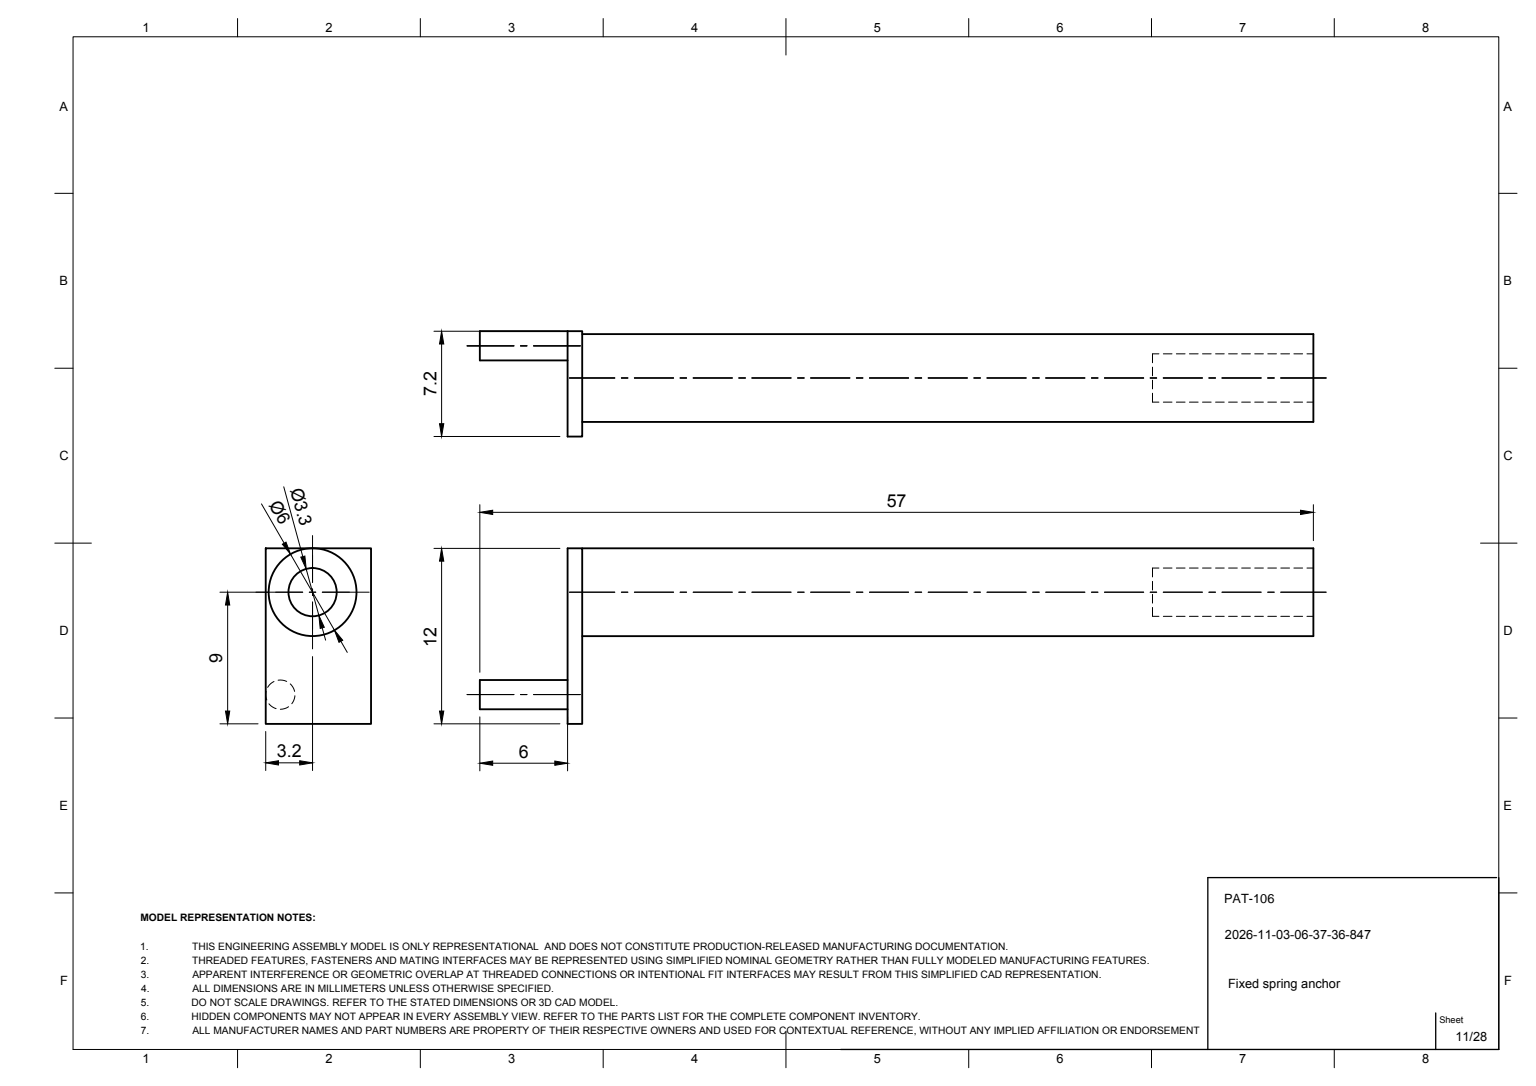
ISO-10303-21;
HEADER;
/* Generated by software containing ST-Developer
 * from STEP Tools, Inc. (www.steptools.com) 
 */

FILE_DESCRIPTION(
/* description */ ('Torsion-spring ratchet demonstrator'),
/* implementation_level */ '2;1');

FILE_NAME(
/* name */ 'Fixed spring anchor.step',
/* time_stamp */ '2026-10-29T17:29:17-07:00',
/* author */ (''),
/* organization */ (''),
/* preprocessor_version */ 'ST-DEVELOPER v20.2',
/* originating_system */ 'Autodesk Translation Framework v15.17.0.0',
/* authorisation */ '');

FILE_SCHEMA (('AUTOMOTIVE_DESIGN { 1 0 10303 214 3 1 1 }'));
ENDSEC;

DATA;
#10=MECHANICAL_DESIGN_GEOMETRIC_PRESENTATION_REPRESENTATION('',(#289),#11258);
#241=SHAPE_REPRESENTATION_RELATIONSHIP('SRR','None',#11367,#265);
#265=ADVANCED_BREP_SHAPE_REPRESENTATION('',(#321),#11237);
#289=STYLED_ITEM('',(#11584),#321);
#321=MANIFOLD_SOLID_BREP('Body1',#5160);
#375=FACE_BOUND('',#1015,.T.);
#461=PLANE('',#5552);
#462=PLANE('',#5557);
#463=PLANE('',#5558);
#464=PLANE('',#5559);
#465=PLANE('',#5562);
#466=PLANE('',#5563);
#467=PLANE('',#5564);
#468=PLANE('',#5565);
#469=PLANE('',#5568);
#668=FACE_OUTER_BOUND('',#1003,.T.);
#669=FACE_OUTER_BOUND('',#1004,.T.);
#670=FACE_OUTER_BOUND('',#1005,.T.);
#671=FACE_OUTER_BOUND('',#1006,.T.);
#672=FACE_OUTER_BOUND('',#1007,.T.);
#673=FACE_OUTER_BOUND('',#1008,.T.);
#674=FACE_OUTER_BOUND('',#1009,.T.);
#675=FACE_OUTER_BOUND('',#1010,.T.);
#676=FACE_OUTER_BOUND('',#1011,.T.);
#677=FACE_OUTER_BOUND('',#1012,.T.);
#678=FACE_OUTER_BOUND('',#1013,.T.);
#679=FACE_OUTER_BOUND('',#1014,.T.);
#1003=EDGE_LOOP('',(#3616,#3617,#3618,#3619));
#1004=EDGE_LOOP('',(#3620));
#1005=EDGE_LOOP('',(#3621,#3622,#3623,#3624,#3625));
#1006=EDGE_LOOP('',(#3626));
#1007=EDGE_LOOP('',(#3627,#3628,#3629,#3630,#3631,#3632,#3633));
#1008=EDGE_LOOP('',(#3634,#3635,#3636,#3637,#3638,#3639,#3640));
#1009=EDGE_LOOP('',(#3641,#3642,#3643,#3644));
#1010=EDGE_LOOP('',(#3645,#3646,#3647,#3648,#3649));
#1011=EDGE_LOOP('',(#3650,#3651,#3652,#3653,#3654));
#1012=EDGE_LOOP('',(#3655,#3656,#3657,#3658));
#1013=EDGE_LOOP('',(#3659,#3660,#3661,#3662,#3663));
#1014=EDGE_LOOP('',(#3664));
#1015=EDGE_LOOP('',(#3665));
#1370=LINE('',#7878,#1753);
#1371=LINE('',#7885,#1754);
#1372=LINE('',#7893,#1755);
#1373=LINE('',#7894,#1756);
#1374=LINE('',#7896,#1757);
#1375=LINE('',#7898,#1758);
#1376=LINE('',#7899,#1759);
#1377=LINE('',#7903,#1760);
#1378=LINE('',#7905,#1761);
#1379=LINE('',#7907,#1762);
#1380=LINE('',#7912,#1763);
#1381=LINE('',#7913,#1764);
#1382=LINE('',#7915,#1765);
#1383=LINE('',#7916,#1766);
#1384=LINE('',#7918,#1767);
#1385=LINE('',#7920,#1768);
#1386=LINE('',#7924,#1769);
#1753=VECTOR('',#6307,0.164999999999999);
#1754=VECTOR('',#6316,0.0999999999999996);
#1755=VECTOR('',#6325,1.);
#1756=VECTOR('',#6326,1.);
#1757=VECTOR('',#6327,1.);
#1758=VECTOR('',#6328,1.);
#1759=VECTOR('',#6329,1.);
#1760=VECTOR('',#6332,1.);
#1761=VECTOR('',#6333,1.);
#1762=VECTOR('',#6334,1.);
#1763=VECTOR('',#6339,1.);
#1764=VECTOR('',#6340,1.);
#1765=VECTOR('',#6343,1.);
#1766=VECTOR('',#6344,1.);
#1767=VECTOR('',#6347,1.);
#1768=VECTOR('',#6350,1.);
#1769=VECTOR('',#6355,0.300000000000001);
#2133=CIRCLE('',#5550,0.164999999999999);
#2134=CIRCLE('',#5551,0.164999999999999);
#2135=CIRCLE('',#5554,0.0999999999999996);
#2136=CIRCLE('',#5555,0.0999999999999996);
#2137=CIRCLE('',#5556,0.0999999999999996);
#2138=CIRCLE('',#5560,0.300000000000001);
#2139=CIRCLE('',#5561,0.300000000000001);
#2140=CIRCLE('',#5567,0.300000000000001);
#2393=VERTEX_POINT('',#7875);
#2394=VERTEX_POINT('',#7877);
#2395=VERTEX_POINT('',#7882);
#2396=VERTEX_POINT('',#7884);
#2397=VERTEX_POINT('',#7886);
#2398=VERTEX_POINT('',#7891);
#2399=VERTEX_POINT('',#7892);
#2400=VERTEX_POINT('',#7895);
#2401=VERTEX_POINT('',#7897);
#2402=VERTEX_POINT('',#7901);
#2403=VERTEX_POINT('',#7902);
#2404=VERTEX_POINT('',#7904);
#2405=VERTEX_POINT('',#7906);
#2406=VERTEX_POINT('',#7908);
#2407=VERTEX_POINT('',#7911);
#2408=VERTEX_POINT('',#7923);
#2868=EDGE_CURVE('',#2393,#2393,#2133,.T.);
#2869=EDGE_CURVE('',#2393,#2394,#1370,.T.);
#2870=EDGE_CURVE('',#2394,#2394,#2134,.T.);
#2871=EDGE_CURVE('',#2395,#2395,#2135,.T.);
#2872=EDGE_CURVE('',#2395,#2396,#1371,.T.);
#2873=EDGE_CURVE('',#2397,#2396,#2136,.T.);
#2874=EDGE_CURVE('',#2396,#2397,#2137,.T.);
#2875=EDGE_CURVE('',#2398,#2399,#1372,.T.);
#2876=EDGE_CURVE('',#2399,#2397,#1373,.T.);
#2877=EDGE_CURVE('',#2397,#2400,#1374,.T.);
#2878=EDGE_CURVE('',#2400,#2401,#1375,.T.);
#2879=EDGE_CURVE('',#2401,#2398,#1376,.T.);
#2880=EDGE_CURVE('',#2402,#2403,#1377,.T.);
#2881=EDGE_CURVE('',#2404,#2402,#1378,.T.);
#2882=EDGE_CURVE('',#2405,#2404,#1379,.T.);
#2883=EDGE_CURVE('',#2405,#2406,#2138,.T.);
#2884=EDGE_CURVE('',#2406,#2405,#2139,.T.);
#2885=EDGE_CURVE('',#2407,#2405,#1380,.T.);
#2886=EDGE_CURVE('',#2403,#2407,#1381,.T.);
#2887=EDGE_CURVE('',#2402,#2398,#1382,.T.);
#2888=EDGE_CURVE('',#2404,#2401,#1383,.T.);
#2889=EDGE_CURVE('',#2407,#2400,#1384,.T.);
#2890=EDGE_CURVE('',#2403,#2399,#1385,.T.);
#2891=EDGE_CURVE('',#2406,#2408,#1386,.T.);
#2892=EDGE_CURVE('',#2408,#2408,#2140,.T.);
#3616=ORIENTED_EDGE('',*,*,#2868,.F.);
#3617=ORIENTED_EDGE('',*,*,#2869,.T.);
#3618=ORIENTED_EDGE('',*,*,#2870,.T.);
#3619=ORIENTED_EDGE('',*,*,#2869,.F.);
#3620=ORIENTED_EDGE('',*,*,#2870,.F.);
#3621=ORIENTED_EDGE('',*,*,#2871,.F.);
#3622=ORIENTED_EDGE('',*,*,#2872,.T.);
#3623=ORIENTED_EDGE('',*,*,#2873,.F.);
#3624=ORIENTED_EDGE('',*,*,#2874,.F.);
#3625=ORIENTED_EDGE('',*,*,#2872,.F.);
#3626=ORIENTED_EDGE('',*,*,#2871,.T.);
#3627=ORIENTED_EDGE('',*,*,#2875,.T.);
#3628=ORIENTED_EDGE('',*,*,#2876,.T.);
#3629=ORIENTED_EDGE('',*,*,#2873,.T.);
#3630=ORIENTED_EDGE('',*,*,#2874,.T.);
#3631=ORIENTED_EDGE('',*,*,#2877,.T.);
#3632=ORIENTED_EDGE('',*,*,#2878,.T.);
#3633=ORIENTED_EDGE('',*,*,#2879,.T.);
#3634=ORIENTED_EDGE('',*,*,#2880,.F.);
#3635=ORIENTED_EDGE('',*,*,#2881,.F.);
#3636=ORIENTED_EDGE('',*,*,#2882,.F.);
#3637=ORIENTED_EDGE('',*,*,#2883,.T.);
#3638=ORIENTED_EDGE('',*,*,#2884,.T.);
#3639=ORIENTED_EDGE('',*,*,#2885,.F.);
#3640=ORIENTED_EDGE('',*,*,#2886,.F.);
#3641=ORIENTED_EDGE('',*,*,#2881,.T.);
#3642=ORIENTED_EDGE('',*,*,#2887,.T.);
#3643=ORIENTED_EDGE('',*,*,#2879,.F.);
#3644=ORIENTED_EDGE('',*,*,#2888,.F.);
#3645=ORIENTED_EDGE('',*,*,#2885,.T.);
#3646=ORIENTED_EDGE('',*,*,#2882,.T.);
#3647=ORIENTED_EDGE('',*,*,#2888,.T.);
#3648=ORIENTED_EDGE('',*,*,#2878,.F.);
#3649=ORIENTED_EDGE('',*,*,#2889,.F.);
#3650=ORIENTED_EDGE('',*,*,#2886,.T.);
#3651=ORIENTED_EDGE('',*,*,#2889,.T.);
#3652=ORIENTED_EDGE('',*,*,#2877,.F.);
#3653=ORIENTED_EDGE('',*,*,#2876,.F.);
#3654=ORIENTED_EDGE('',*,*,#2890,.F.);
#3655=ORIENTED_EDGE('',*,*,#2880,.T.);
#3656=ORIENTED_EDGE('',*,*,#2890,.T.);
#3657=ORIENTED_EDGE('',*,*,#2875,.F.);
#3658=ORIENTED_EDGE('',*,*,#2887,.F.);
#3659=ORIENTED_EDGE('',*,*,#2883,.F.);
#3660=ORIENTED_EDGE('',*,*,#2884,.F.);
#3661=ORIENTED_EDGE('',*,*,#2891,.T.);
#3662=ORIENTED_EDGE('',*,*,#2892,.T.);
#3663=ORIENTED_EDGE('',*,*,#2891,.F.);
#3664=ORIENTED_EDGE('',*,*,#2892,.F.);
#3665=ORIENTED_EDGE('',*,*,#2868,.T.);
#4785=CYLINDRICAL_SURFACE('',#5549,0.164999999999999);
#4786=CYLINDRICAL_SURFACE('',#5553,0.0999999999999996);
#4787=CYLINDRICAL_SURFACE('',#5566,0.300000000000001);
#4894=ADVANCED_FACE('',(#668),#4785,.F.);
#4895=ADVANCED_FACE('',(#669),#461,.F.);
#4896=ADVANCED_FACE('',(#670),#4786,.T.);
#4897=ADVANCED_FACE('',(#671),#462,.T.);
#4898=ADVANCED_FACE('',(#672),#463,.T.);
#4899=ADVANCED_FACE('',(#673),#464,.F.);
#4900=ADVANCED_FACE('',(#674),#465,.T.);
#4901=ADVANCED_FACE('',(#675),#466,.T.);
#4902=ADVANCED_FACE('',(#676),#467,.T.);
#4903=ADVANCED_FACE('',(#677),#468,.T.);
#4904=ADVANCED_FACE('',(#678),#4787,.T.);
#4905=ADVANCED_FACE('',(#679,#375),#469,.F.);
#5160=CLOSED_SHELL('',(#4894,#4895,#4896,#4897,#4898,#4899,#4900,#4901,
#4902,#4903,#4904,#4905));
#5548=AXIS2_PLACEMENT_3D('',#7873,#6301,#6302);
#5549=AXIS2_PLACEMENT_3D('',#7874,#6303,#6304);
#5550=AXIS2_PLACEMENT_3D('',#7876,#6305,#6306);
#5551=AXIS2_PLACEMENT_3D('',#7879,#6308,#6309);
#5552=AXIS2_PLACEMENT_3D('',#7880,#6310,#6311);
#5553=AXIS2_PLACEMENT_3D('',#7881,#6312,#6313);
#5554=AXIS2_PLACEMENT_3D('',#7883,#6314,#6315);
#5555=AXIS2_PLACEMENT_3D('',#7887,#6317,#6318);
#5556=AXIS2_PLACEMENT_3D('',#7888,#6319,#6320);
#5557=AXIS2_PLACEMENT_3D('',#7889,#6321,#6322);
#5558=AXIS2_PLACEMENT_3D('',#7890,#6323,#6324);
#5559=AXIS2_PLACEMENT_3D('',#7900,#6330,#6331);
#5560=AXIS2_PLACEMENT_3D('',#7909,#6335,#6336);
#5561=AXIS2_PLACEMENT_3D('',#7910,#6337,#6338);
#5562=AXIS2_PLACEMENT_3D('',#7914,#6341,#6342);
#5563=AXIS2_PLACEMENT_3D('',#7917,#6345,#6346);
#5564=AXIS2_PLACEMENT_3D('',#7919,#6348,#6349);
#5565=AXIS2_PLACEMENT_3D('',#7921,#6351,#6352);
#5566=AXIS2_PLACEMENT_3D('',#7922,#6353,#6354);
#5567=AXIS2_PLACEMENT_3D('',#7925,#6356,#6357);
#5568=AXIS2_PLACEMENT_3D('',#7926,#6358,#6359);
#6301=DIRECTION('axis',(0.,0.,1.));
#6302=DIRECTION('refdir',(1.,0.,0.));
#6303=DIRECTION('center_axis',(0.,0.,1.));
#6304=DIRECTION('ref_axis',(1.,0.,0.));
#6305=DIRECTION('center_axis',(0.,0.,1.));
#6306=DIRECTION('ref_axis',(1.,0.,0.));
#6307=DIRECTION('',(0.,0.,1.));
#6308=DIRECTION('center_axis',(0.,0.,1.));
#6309=DIRECTION('ref_axis',(1.,0.,0.));
#6310=DIRECTION('center_axis',(0.,0.,1.));
#6311=DIRECTION('ref_axis',(1.,0.,0.));
#6312=DIRECTION('center_axis',(0.,0.,1.));
#6313=DIRECTION('ref_axis',(1.,0.,0.));
#6314=DIRECTION('center_axis',(0.,0.,1.));
#6315=DIRECTION('ref_axis',(1.,0.,0.));
#6316=DIRECTION('',(0.,0.,-1.));
#6317=DIRECTION('center_axis',(0.,0.,-1.));
#6318=DIRECTION('ref_axis',(1.,0.,0.));
#6319=DIRECTION('center_axis',(0.,0.,-1.));
#6320=DIRECTION('ref_axis',(1.,0.,0.));
#6321=DIRECTION('center_axis',(0.,0.,1.));
#6322=DIRECTION('ref_axis',(1.,0.,0.));
#6323=DIRECTION('center_axis',(0.,0.,1.));
#6324=DIRECTION('ref_axis',(1.,0.,0.));
#6325=DIRECTION('',(0.,-1.,0.));
#6326=DIRECTION('',(1.,0.,0.));
#6327=DIRECTION('',(1.,0.,0.));
#6328=DIRECTION('',(0.,1.,0.));
#6329=DIRECTION('',(-1.,0.,0.));
#6330=DIRECTION('center_axis',(0.,0.,1.));
#6331=DIRECTION('ref_axis',(1.,0.,0.));
#6332=DIRECTION('',(0.,-1.,0.));
#6333=DIRECTION('',(-1.,0.,0.));
#6334=DIRECTION('',(0.,1.,0.));
#6335=DIRECTION('center_axis',(0.,0.,1.));
#6336=DIRECTION('ref_axis',(1.,0.,0.));
#6337=DIRECTION('center_axis',(0.,0.,1.));
#6338=DIRECTION('ref_axis',(1.,0.,0.));
#6339=DIRECTION('',(0.,1.,0.));
#6340=DIRECTION('',(1.,0.,0.));
#6341=DIRECTION('center_axis',(0.,1.,0.));
#6342=DIRECTION('ref_axis',(-1.,0.,0.));
#6343=DIRECTION('',(0.,0.,1.));
#6344=DIRECTION('',(0.,0.,1.));
#6345=DIRECTION('center_axis',(1.,0.,0.));
#6346=DIRECTION('ref_axis',(0.,1.,0.));
#6347=DIRECTION('',(0.,0.,1.));
#6348=DIRECTION('center_axis',(0.,-1.,0.));
#6349=DIRECTION('ref_axis',(1.,0.,0.));
#6350=DIRECTION('',(0.,0.,1.));
#6351=DIRECTION('center_axis',(-1.,0.,0.));
#6352=DIRECTION('ref_axis',(0.,-1.,0.));
#6353=DIRECTION('center_axis',(0.,0.,1.));
#6354=DIRECTION('ref_axis',(1.,0.,0.));
#6355=DIRECTION('',(0.,0.,-1.));
#6356=DIRECTION('center_axis',(0.,0.,1.));
#6357=DIRECTION('ref_axis',(1.,0.,0.));
#6358=DIRECTION('center_axis',(0.,0.,1.));
#6359=DIRECTION('ref_axis',(1.,0.,0.));
#7873=CARTESIAN_POINT('',(0.,0.,0.));
#7874=CARTESIAN_POINT('Origin',(8.8,-2.47,0.9));
#7875=CARTESIAN_POINT('',(8.635,-2.47,1.));
#7876=CARTESIAN_POINT('Origin',(8.8,-2.47,1.));
#7877=CARTESIAN_POINT('',(8.635,-2.47,2.1));
#7878=CARTESIAN_POINT('',(8.635,-2.47,0.9));
#7879=CARTESIAN_POINT('Origin',(8.8,-2.47,2.1));
#7880=CARTESIAN_POINT('Origin',(8.8,-2.47,2.1));
#7881=CARTESIAN_POINT('Origin',(8.1,-2.69,6.1));
#7882=CARTESIAN_POINT('',(8.,-2.69,6.7));
#7883=CARTESIAN_POINT('Origin',(8.1,-2.69,6.7));
#7884=CARTESIAN_POINT('',(8.,-2.69,6.1));
#7885=CARTESIAN_POINT('',(8.,-2.69,6.1));
#7886=CARTESIAN_POINT('',(8.1,-2.79,6.1));
#7887=CARTESIAN_POINT('Origin',(8.1,-2.69,6.1));
#7888=CARTESIAN_POINT('Origin',(8.1,-2.69,6.1));
#7889=CARTESIAN_POINT('Origin',(8.1,-2.69,6.7));
#7890=CARTESIAN_POINT('Origin',(8.5,-2.43,6.1));
#7891=CARTESIAN_POINT('',(7.9,-2.07,6.1));
#7892=CARTESIAN_POINT('',(7.9,-2.79,6.1));
#7893=CARTESIAN_POINT('',(7.9,-2.07,6.1));
#7894=CARTESIAN_POINT('',(7.9,-2.79,6.1));
#7895=CARTESIAN_POINT('',(9.1,-2.79,6.1));
#7896=CARTESIAN_POINT('',(7.9,-2.79,6.1));
#7897=CARTESIAN_POINT('',(9.1,-2.07,6.1));
#7898=CARTESIAN_POINT('',(9.1,-2.79,6.1));
#7899=CARTESIAN_POINT('',(9.1,-2.07,6.1));
#7900=CARTESIAN_POINT('Origin',(8.5,-2.43,6.));
#7901=CARTESIAN_POINT('',(7.9,-2.07,6.));
#7902=CARTESIAN_POINT('',(7.9,-2.79,6.));
#7903=CARTESIAN_POINT('',(7.9,-2.07,6.));
#7904=CARTESIAN_POINT('',(9.1,-2.07,6.));
#7905=CARTESIAN_POINT('',(9.1,-2.07,6.));
#7906=CARTESIAN_POINT('',(9.1,-2.47,6.));
#7907=CARTESIAN_POINT('',(9.1,-2.79,6.));
#7908=CARTESIAN_POINT('',(8.5,-2.47,6.));
#7909=CARTESIAN_POINT('Origin',(8.8,-2.47,6.));
#7910=CARTESIAN_POINT('Origin',(8.8,-2.47,6.));
#7911=CARTESIAN_POINT('',(9.1,-2.79,6.));
#7912=CARTESIAN_POINT('',(9.1,-2.79,6.));
#7913=CARTESIAN_POINT('',(7.9,-2.79,6.));
#7914=CARTESIAN_POINT('Origin',(9.1,-2.07,6.));
#7915=CARTESIAN_POINT('',(7.9,-2.07,6.));
#7916=CARTESIAN_POINT('',(9.1,-2.07,6.));
#7917=CARTESIAN_POINT('Origin',(9.1,-2.79,6.));
#7918=CARTESIAN_POINT('',(9.1,-2.79,6.));
#7919=CARTESIAN_POINT('Origin',(7.9,-2.79,6.));
#7920=CARTESIAN_POINT('',(7.9,-2.79,6.));
#7921=CARTESIAN_POINT('Origin',(7.9,-2.07,6.));
#7922=CARTESIAN_POINT('Origin',(8.8,-2.47,1.));
#7923=CARTESIAN_POINT('',(8.5,-2.47,1.));
#7924=CARTESIAN_POINT('',(8.5,-2.47,1.));
#7925=CARTESIAN_POINT('Origin',(8.8,-2.47,1.));
#7926=CARTESIAN_POINT('Origin',(8.8,-2.47,1.));
#11207=UNCERTAINTY_MEASURE_WITH_UNIT(LENGTH_MEASURE(0.001),#11259,
'DISTANCE_ACCURACY_VALUE',
'Maximum model space distance between geometric entities at asserted c
onnectivities');
#11228=UNCERTAINTY_MEASURE_WITH_UNIT(LENGTH_MEASURE(0.001),#11259,
'DISTANCE_ACCURACY_VALUE',
'Maximum model space distance between geometric entities at asserted c
onnectivities');
#11237=(
GEOMETRIC_REPRESENTATION_CONTEXT(3)
GLOBAL_UNCERTAINTY_ASSIGNED_CONTEXT((#11207))
GLOBAL_UNIT_ASSIGNED_CONTEXT((#11259,#11261,#11262))
REPRESENTATION_CONTEXT('','3D')
);
#11258=(
GEOMETRIC_REPRESENTATION_CONTEXT(3)
GLOBAL_UNCERTAINTY_ASSIGNED_CONTEXT((#11228))
GLOBAL_UNIT_ASSIGNED_CONTEXT((#11259,#11261,#11262))
REPRESENTATION_CONTEXT('','3D')
);
#11259=(
LENGTH_UNIT()
NAMED_UNIT(*)
SI_UNIT(.CENTI.,.METRE.)
);
#11261=(
NAMED_UNIT(*)
PLANE_ANGLE_UNIT()
SI_UNIT($,.RADIAN.)
);
#11262=(
NAMED_UNIT(*)
SI_UNIT($,.STERADIAN.)
SOLID_ANGLE_UNIT()
);
#11271=SHAPE_DEFINITION_REPRESENTATION(#11300,#11367);
#11300=PRODUCT_DEFINITION_SHAPE('',$,#11397);
#11367=SHAPE_REPRESENTATION('',(#5548),#11237);
#11388=PRODUCT_DEFINITION_CONTEXT('part definition',#11477,'design');
#11397=PRODUCT_DEFINITION('Fixed spring anchor','Fixed spring anchor',#11426,
#11388);
#11426=PRODUCT_DEFINITION_FORMATION('',$,#11487);
#11477=APPLICATION_CONTEXT(
'Core Data for Automotive Mechanical Design Process');
#11478=PRODUCT_CONTEXT('part definition',#11477,'mechanical');
#11487=PRODUCT('Fixed spring anchor','Fixed spring anchor',
'Fixed spring anchor',(#11478));
#11578=COLOUR_RGB('Grey',0.48,0.52,0.57);
#11579=FILL_AREA_STYLE_COLOUR('',#11578);
#11580=FILL_AREA_STYLE('',(#11579));
#11581=SURFACE_STYLE_FILL_AREA(#11580);
#11582=SURFACE_SIDE_STYLE('',(#11581));
#11583=SURFACE_STYLE_USAGE(.BOTH.,#11582);
#11584=PRESENTATION_STYLE_ASSIGNMENT((#11583));
ENDSEC;
END-ISO-10303-21;
